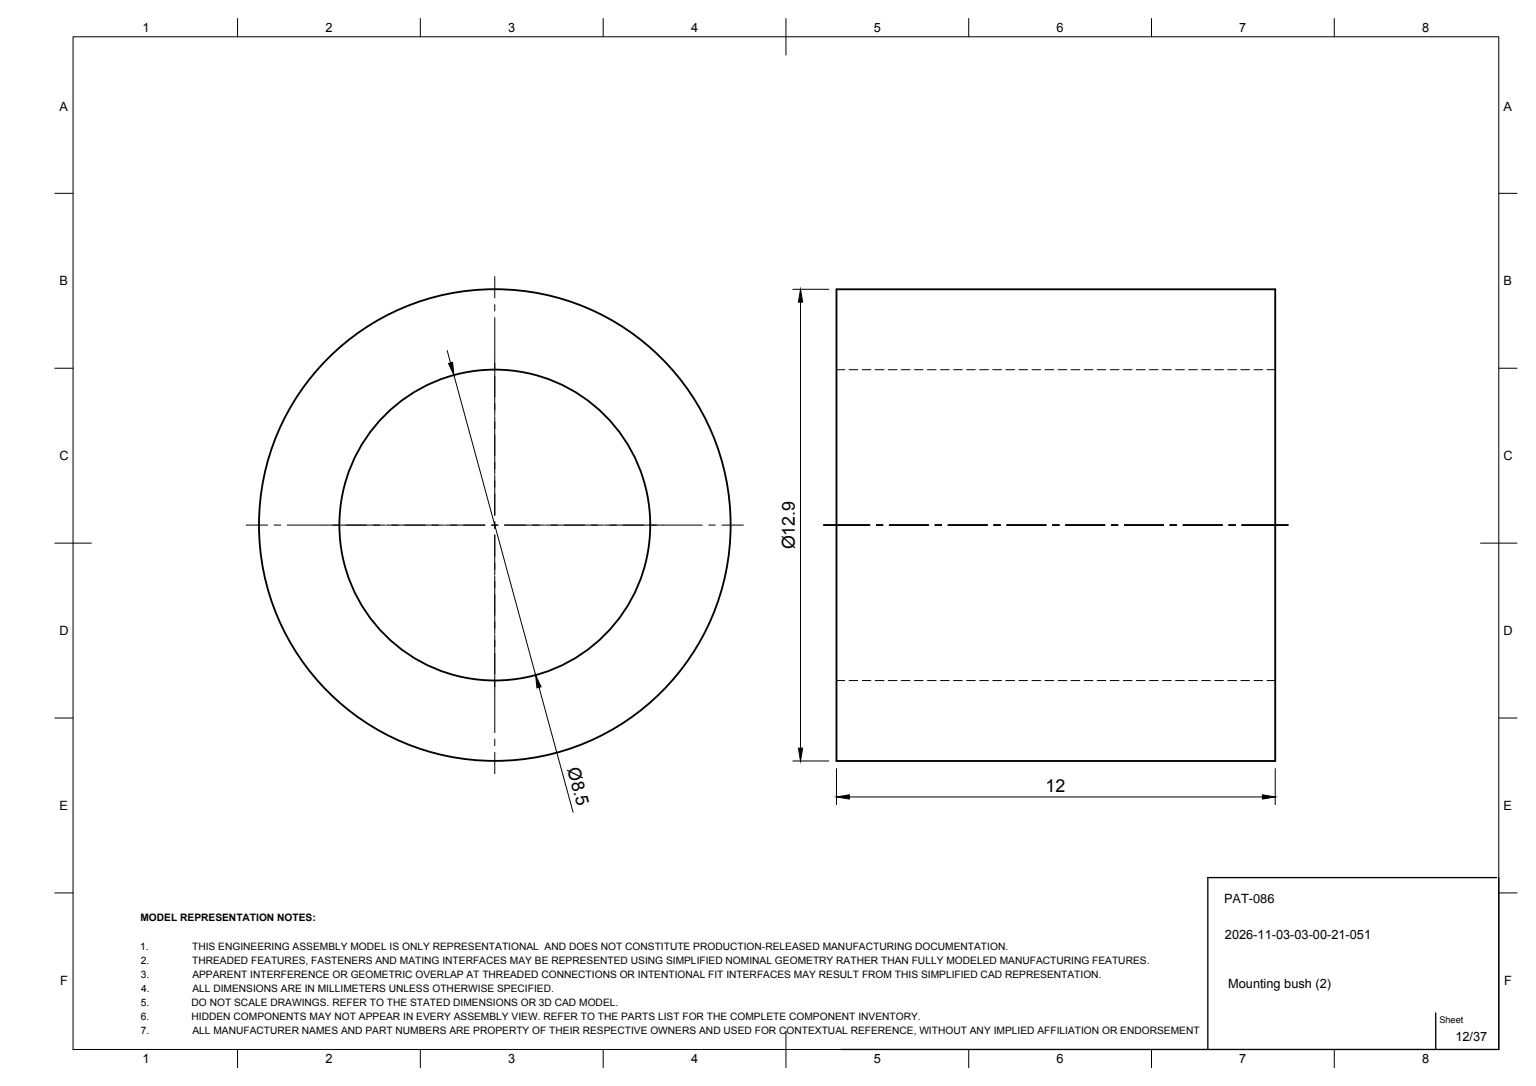
ISO-10303-21;
HEADER;
/* Generated by software containing ST-Developer
 * from STEP Tools, Inc. (www.steptools.com) 
 */

FILE_DESCRIPTION(
/* description */ ('Ratchet and pawl hand winch drum'),
/* implementation_level */ '2;1');

FILE_NAME(
/* name */ 'Mounting bush (2).step',
/* time_stamp */ '2026-10-27T12:42:58-07:00',
/* author */ (''),
/* organization */ (''),
/* preprocessor_version */ 'ST-DEVELOPER v20.2',
/* originating_system */ 'Autodesk Translation Framework v15.17.0.0',
/* authorisation */ '');

FILE_SCHEMA (('AUTOMOTIVE_DESIGN { 1 0 10303 214 3 1 1 }'));
ENDSEC;

DATA;
#10=MECHANICAL_DESIGN_GEOMETRIC_PRESENTATION_REPRESENTATION('',(#396),#11801);
#328=SHAPE_REPRESENTATION_RELATIONSHIP('SRR','None',#11954,#362);
#362=ADVANCED_BREP_SHAPE_REPRESENTATION('',(#431),#11771);
#396=STYLED_ITEM('',(#12206),#431);
#431=MANIFOLD_SOLID_BREP('Body1',#6273);
#512=FACE_BOUND('',#1331,.T.);
#513=FACE_BOUND('',#1333,.T.);
#643=PLANE('',#6839);
#644=PLANE('',#6840);
#916=FACE_OUTER_BOUND('',#1328,.T.);
#917=FACE_OUTER_BOUND('',#1329,.T.);
#918=FACE_OUTER_BOUND('',#1330,.T.);
#919=FACE_OUTER_BOUND('',#1332,.T.);
#1328=EDGE_LOOP('',(#4571,#4572,#4573,#4574));
#1329=EDGE_LOOP('',(#4575,#4576,#4577,#4578));
#1330=EDGE_LOOP('',(#4579));
#1331=EDGE_LOOP('',(#4580));
#1332=EDGE_LOOP('',(#4581));
#1333=EDGE_LOOP('',(#4582));
#1791=LINE('',#9587,#2302);
#1792=LINE('',#9593,#2303);
#2302=VECTOR('',#7764,0.425);
#2303=VECTOR('',#7771,0.645);
#2787=CIRCLE('',#6834,0.425);
#2788=CIRCLE('',#6835,0.425);
#2789=CIRCLE('',#6837,0.645);
#2790=CIRCLE('',#6838,0.645);
#3050=VERTEX_POINT('',#9584);
#3051=VERTEX_POINT('',#9586);
#3052=VERTEX_POINT('',#9590);
#3053=VERTEX_POINT('',#9592);
#3629=EDGE_CURVE('',#3050,#3050,#2787,.T.);
#3630=EDGE_CURVE('',#3050,#3051,#1791,.T.);
#3631=EDGE_CURVE('',#3051,#3051,#2788,.T.);
#3632=EDGE_CURVE('',#3052,#3052,#2789,.T.);
#3633=EDGE_CURVE('',#3052,#3053,#1792,.T.);
#3634=EDGE_CURVE('',#3053,#3053,#2790,.T.);
#4571=ORIENTED_EDGE('',*,*,#3629,.F.);
#4572=ORIENTED_EDGE('',*,*,#3630,.T.);
#4573=ORIENTED_EDGE('',*,*,#3631,.T.);
#4574=ORIENTED_EDGE('',*,*,#3630,.F.);
#4575=ORIENTED_EDGE('',*,*,#3632,.F.);
#4576=ORIENTED_EDGE('',*,*,#3633,.T.);
#4577=ORIENTED_EDGE('',*,*,#3634,.T.);
#4578=ORIENTED_EDGE('',*,*,#3633,.F.);
#4579=ORIENTED_EDGE('',*,*,#3632,.T.);
#4580=ORIENTED_EDGE('',*,*,#3629,.T.);
#4581=ORIENTED_EDGE('',*,*,#3634,.F.);
#4582=ORIENTED_EDGE('',*,*,#3631,.F.);
#5841=CYLINDRICAL_SURFACE('',#6833,0.425);
#5842=CYLINDRICAL_SURFACE('',#6836,0.645);
#5986=ADVANCED_FACE('',(#916),#5841,.F.);
#5987=ADVANCED_FACE('',(#917),#5842,.T.);
#5988=ADVANCED_FACE('',(#918,#512),#643,.T.);
#5989=ADVANCED_FACE('',(#919,#513),#644,.F.);
#6273=CLOSED_SHELL('',(#5986,#5987,#5988,#5989));
#6832=AXIS2_PLACEMENT_3D('',#9582,#7758,#7759);
#6833=AXIS2_PLACEMENT_3D('',#9583,#7760,#7761);
#6834=AXIS2_PLACEMENT_3D('',#9585,#7762,#7763);
#6835=AXIS2_PLACEMENT_3D('',#9588,#7765,#7766);
#6836=AXIS2_PLACEMENT_3D('',#9589,#7767,#7768);
#6837=AXIS2_PLACEMENT_3D('',#9591,#7769,#7770);
#6838=AXIS2_PLACEMENT_3D('',#9594,#7772,#7773);
#6839=AXIS2_PLACEMENT_3D('',#9595,#7774,#7775);
#6840=AXIS2_PLACEMENT_3D('',#9596,#7776,#7777);
#7758=DIRECTION('axis',(0.,0.,1.));
#7759=DIRECTION('refdir',(1.,0.,0.));
#7760=DIRECTION('center_axis',(0.,0.,1.));
#7761=DIRECTION('ref_axis',(1.,0.,0.));
#7762=DIRECTION('center_axis',(0.,0.,-1.));
#7763=DIRECTION('ref_axis',(1.,0.,0.));
#7764=DIRECTION('',(0.,0.,-1.));
#7765=DIRECTION('center_axis',(0.,0.,-1.));
#7766=DIRECTION('ref_axis',(1.,0.,0.));
#7767=DIRECTION('center_axis',(0.,0.,1.));
#7768=DIRECTION('ref_axis',(1.,0.,0.));
#7769=DIRECTION('center_axis',(0.,0.,1.));
#7770=DIRECTION('ref_axis',(1.,0.,0.));
#7771=DIRECTION('',(0.,0.,-1.));
#7772=DIRECTION('center_axis',(0.,0.,1.));
#7773=DIRECTION('ref_axis',(1.,0.,0.));
#7774=DIRECTION('center_axis',(0.,0.,1.));
#7775=DIRECTION('ref_axis',(1.,0.,0.));
#7776=DIRECTION('center_axis',(0.,0.,1.));
#7777=DIRECTION('ref_axis',(1.,0.,0.));
#9582=CARTESIAN_POINT('',(0.,0.,0.));
#9583=CARTESIAN_POINT('Origin',(-4.75,16.,3.2));
#9584=CARTESIAN_POINT('',(-5.175,16.,4.4));
#9585=CARTESIAN_POINT('Origin',(-4.75,16.,4.4));
#9586=CARTESIAN_POINT('',(-5.175,16.,3.2));
#9587=CARTESIAN_POINT('',(-5.175,16.,3.2));
#9588=CARTESIAN_POINT('Origin',(-4.75,16.,3.2));
#9589=CARTESIAN_POINT('Origin',(-4.75,16.,3.2));
#9590=CARTESIAN_POINT('',(-5.395,16.,4.4));
#9591=CARTESIAN_POINT('Origin',(-4.75,16.,4.4));
#9592=CARTESIAN_POINT('',(-5.395,16.,3.2));
#9593=CARTESIAN_POINT('',(-5.395,16.,3.2));
#9594=CARTESIAN_POINT('Origin',(-4.75,16.,3.2));
#9595=CARTESIAN_POINT('Origin',(-4.75,16.,4.4));
#9596=CARTESIAN_POINT('Origin',(-4.75,16.,3.2));
#11731=UNCERTAINTY_MEASURE_WITH_UNIT(LENGTH_MEASURE(0.001),#11802,
'DISTANCE_ACCURACY_VALUE',
'Maximum model space distance between geometric entities at asserted c
onnectivities');
#11761=UNCERTAINTY_MEASURE_WITH_UNIT(LENGTH_MEASURE(0.001),#11802,
'DISTANCE_ACCURACY_VALUE',
'Maximum model space distance between geometric entities at asserted c
onnectivities');
#11771=(
GEOMETRIC_REPRESENTATION_CONTEXT(3)
GLOBAL_UNCERTAINTY_ASSIGNED_CONTEXT((#11731))
GLOBAL_UNIT_ASSIGNED_CONTEXT((#11802,#11804,#11805))
REPRESENTATION_CONTEXT('','3D')
);
#11801=(
GEOMETRIC_REPRESENTATION_CONTEXT(3)
GLOBAL_UNCERTAINTY_ASSIGNED_CONTEXT((#11761))
GLOBAL_UNIT_ASSIGNED_CONTEXT((#11802,#11804,#11805))
REPRESENTATION_CONTEXT('','3D')
);
#11802=(
LENGTH_UNIT()
NAMED_UNIT(*)
SI_UNIT(.CENTI.,.METRE.)
);
#11804=(
NAMED_UNIT(*)
PLANE_ANGLE_UNIT()
SI_UNIT($,.RADIAN.)
);
#11805=(
NAMED_UNIT(*)
SI_UNIT($,.STERADIAN.)
SOLID_ANGLE_UNIT()
);
#11815=SHAPE_DEFINITION_REPRESENTATION(#11854,#11954);
#11854=PRODUCT_DEFINITION_SHAPE('',$,#11994);
#11954=SHAPE_REPRESENTATION('',(#6832),#11771);
#11984=PRODUCT_DEFINITION_CONTEXT('part definition',#12103,'design');
#11994=PRODUCT_DEFINITION('Mounting bush (2)','Mounting bush (2)',#12033,
#11984);
#12033=PRODUCT_DEFINITION_FORMATION('',$,#12114);
#12103=APPLICATION_CONTEXT(
'Core Data for Automotive Mechanical Design Process');
#12104=PRODUCT_CONTEXT('part definition',#12103,'mechanical');
#12114=PRODUCT('Mounting bush (2)','Mounting bush (2)','Mounting bush (2)',(#12104));
#12200=COLOUR_RGB('Sky Blue',0.24,0.69,0.87);
#12201=FILL_AREA_STYLE_COLOUR('',#12200);
#12202=FILL_AREA_STYLE('',(#12201));
#12203=SURFACE_STYLE_FILL_AREA(#12202);
#12204=SURFACE_SIDE_STYLE('',(#12203));
#12205=SURFACE_STYLE_USAGE(.BOTH.,#12204);
#12206=PRESENTATION_STYLE_ASSIGNMENT((#12205));
ENDSEC;
END-ISO-10303-21;
